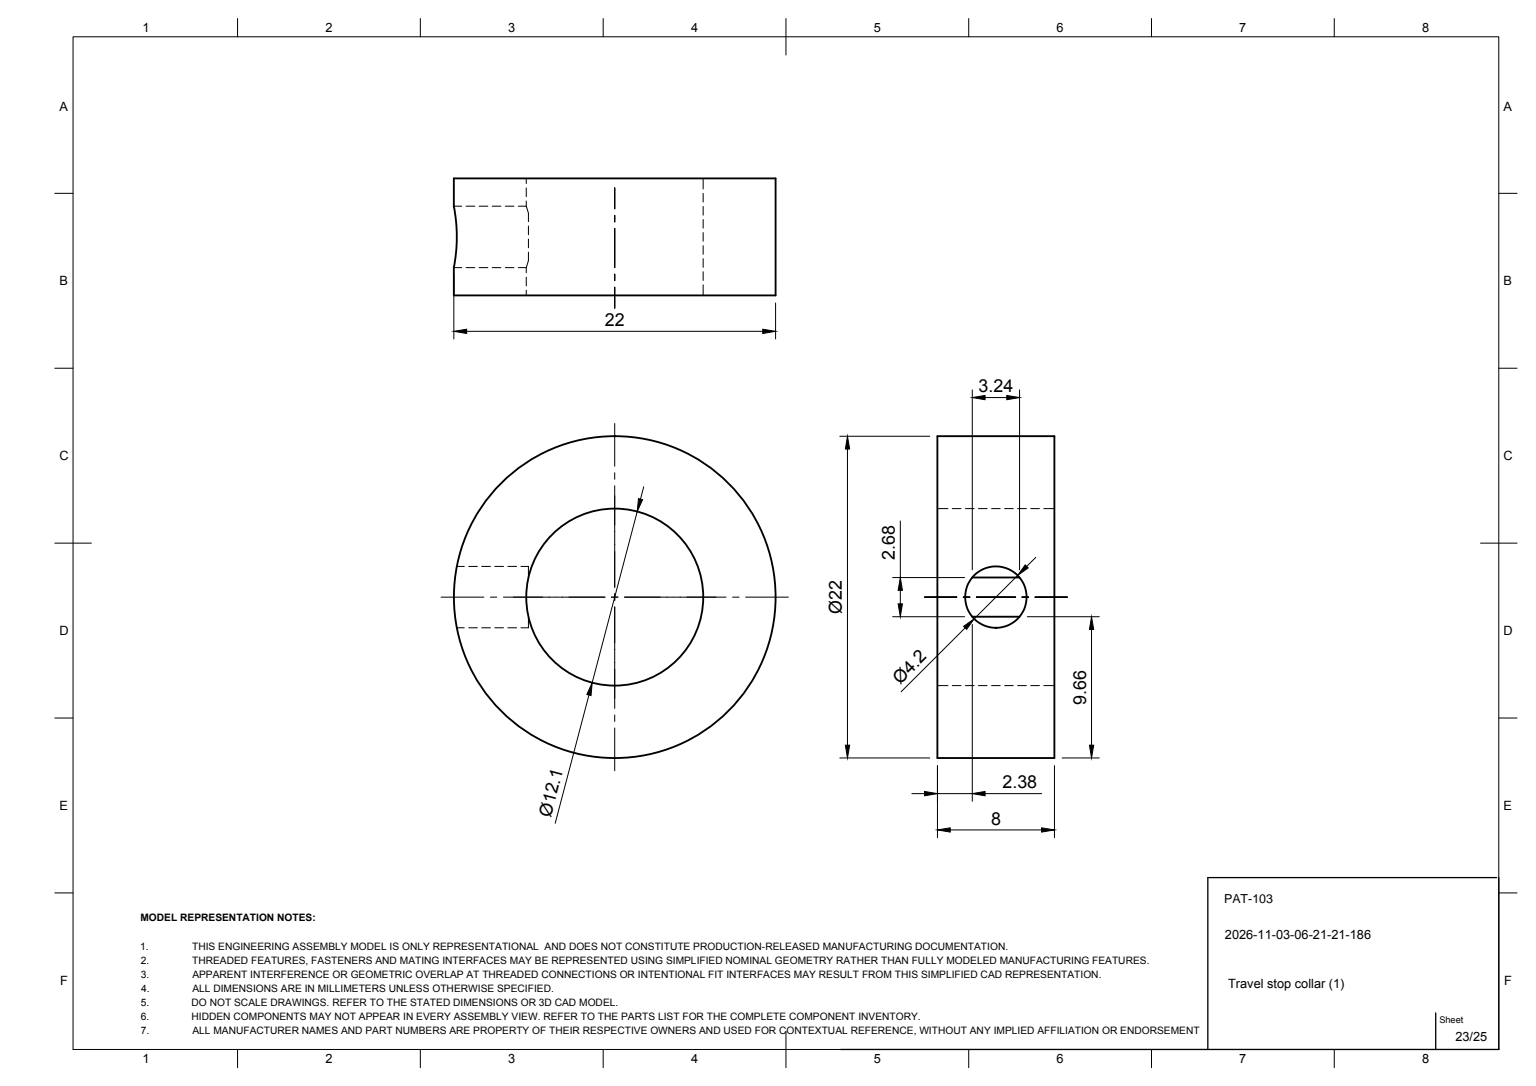
ISO-10303-21;
HEADER;
/* Generated by software containing ST-Developer
 * from STEP Tools, Inc. (www.steptools.com) 
 */

FILE_DESCRIPTION(
/* description */ ('Telescoping shaft support with lock collar'),
/* implementation_level */ '2;1');

FILE_NAME(
/* name */ 'Travel stop collar (1).step',
/* time_stamp */ '2026-10-27T10:48:51-07:00',
/* author */ (''),
/* organization */ (''),
/* preprocessor_version */ 'ST-DEVELOPER v20.2',
/* originating_system */ 'Autodesk Translation Framework v15.17.0.0',
/* authorisation */ '');

FILE_SCHEMA (('AUTOMOTIVE_DESIGN { 1 0 10303 214 3 1 1 }'));
ENDSEC;

DATA;
#10=MECHANICAL_DESIGN_GEOMETRIC_PRESENTATION_REPRESENTATION('',(#256),#7349);
#194=B_SPLINE_CURVE_WITH_KNOTS('',3,(#7006,#7007,#7008,#7009,#7010,#7011),
 .UNSPECIFIED.,.F.,.F.,(4,2,4),(0.81808890434917,0.878131747417167,0.957937926194039),
 .UNSPECIFIED.);
#195=B_SPLINE_CURVE_WITH_KNOTS('',3,(#7015,#7016,#7017,#7018,#7019,#7020),
 .UNSPECIFIED.,.F.,.F.,(4,2,4),(0.31931264206468,0.399118820841551,0.459161663909546),
 .UNSPECIFIED.);
#196=B_SPLINE_CURVE_WITH_KNOTS('',3,(#7021,#7022,#7023,#7024,#7025,#7026),
 .UNSPECIFIED.,.F.,.F.,(4,2,4),(0.179463620219813,0.239506463287808,0.31931264206468),
 .UNSPECIFIED.);
#197=B_SPLINE_CURVE_WITH_KNOTS('',3,(#7027,#7028,#7029,#7030,#7031,#7032),
 .UNSPECIFIED.,.F.,.F.,(4,2,4),(0.957937926194039,1.03774410497091,1.09778694803891),
 .UNSPECIFIED.);
#198=B_SPLINE_CURVE_WITH_KNOTS('',3,(#7036,#7037,#7038,#7039,#7040,#7041,
#7042,#7043,#7044,#7045),.UNSPECIFIED.,.F.,.F.,(4,2,2,2,4),(0.,0.0793157643915219,
0.158631528783044,0.23794361593365,0.317255703084256),.UNSPECIFIED.);
#199=B_SPLINE_CURVE_WITH_KNOTS('',3,(#7047,#7048,#7049,#7050,#7051,#7052,
#7053,#7054,#7055,#7056),.UNSPECIFIED.,.F.,.F.,(4,2,2,2,4),(0.951767109252769,
1.03107919640337,1.11039128355398,1.1897070479455,1.26902281233703),
 .UNSPECIFIED.);
#200=B_SPLINE_CURVE_WITH_KNOTS('',3,(#7057,#7058,#7059,#7060,#7061,#7062,
#7063,#7064,#7065,#7066,#7067,#7068,#7069,#7070,#7071,#7072,#7073,#7074),
 .UNSPECIFIED.,.F.,.F.,(4,2,2,2,2,2,2,2,4),(0.317255703084256,0.396567790234863,
0.475879877385469,0.555195641776991,0.634511406168513,0.713827170560035,
0.793142934951556,0.872455022102163,0.951767109252769),.UNSPECIFIED.);
#216=SHAPE_REPRESENTATION_RELATIONSHIP('SRR','None',#7460,#236);
#236=ADVANCED_BREP_SHAPE_REPRESENTATION('',(#275),#7344);
#256=STYLED_ITEM('',(#7641),#275);
#275=MANIFOLD_SOLID_BREP('Body1',#3980);
#351=FACE_BOUND('',#976,.T.);
#352=FACE_BOUND('',#978,.T.);
#465=PLANE('',#4587);
#466=PLANE('',#4591);
#467=PLANE('',#4598);
#468=PLANE('',#4599);
#672=FACE_OUTER_BOUND('',#970,.T.);
#673=FACE_OUTER_BOUND('',#971,.T.);
#674=FACE_OUTER_BOUND('',#972,.T.);
#675=FACE_OUTER_BOUND('',#973,.T.);
#676=FACE_OUTER_BOUND('',#974,.T.);
#677=FACE_OUTER_BOUND('',#975,.T.);
#678=FACE_OUTER_BOUND('',#977,.T.);
#970=EDGE_LOOP('',(#3468,#3469));
#971=EDGE_LOOP('',(#3470,#3471,#3472,#3473,#3474,#3475,#3476,#3477,#3478,
#3479,#3480));
#972=EDGE_LOOP('',(#3481,#3482));
#973=EDGE_LOOP('',(#3483,#3484,#3485,#3486,#3487,#3488,#3489,#3490,#3491,
#3492,#3493,#3494));
#974=EDGE_LOOP('',(#3495,#3496,#3497,#3498,#3499,#3500,#3501,#3502,#3503));
#975=EDGE_LOOP('',(#3504));
#976=EDGE_LOOP('',(#3505));
#977=EDGE_LOOP('',(#3506));
#978=EDGE_LOOP('',(#3507));
#1248=LINE('',#7001,#1528);
#1249=LINE('',#7034,#1529);
#1250=LINE('',#7076,#1530);
#1251=LINE('',#7080,#1531);
#1252=LINE('',#7082,#1532);
#1253=LINE('',#7087,#1533);
#1254=LINE('',#7089,#1534);
#1528=VECTOR('',#5690,1.);
#1529=VECTOR('',#5697,0.210000000000001);
#1530=VECTOR('',#5700,1.);
#1531=VECTOR('',#5705,0.605);
#1532=VECTOR('',#5706,0.605);
#1533=VECTOR('',#5713,1.1);
#1534=VECTOR('',#5714,1.1);
#1768=CIRCLE('',#4588,0.210000000000001);
#1769=CIRCLE('',#4590,0.210000000000001);
#1770=CIRCLE('',#4593,0.605);
#1771=CIRCLE('',#4594,0.605);
#1772=CIRCLE('',#4596,1.1);
#1773=CIRCLE('',#4597,1.1);
#2072=VERTEX_POINT('',#6999);
#2073=VERTEX_POINT('',#7000);
#2074=VERTEX_POINT('',#7004);
#2075=VERTEX_POINT('',#7005);
#2076=VERTEX_POINT('',#7012);
#2077=VERTEX_POINT('',#7014);
#2078=VERTEX_POINT('',#7033);
#2079=VERTEX_POINT('',#7035);
#2080=VERTEX_POINT('',#7046);
#2081=VERTEX_POINT('',#7078);
#2082=VERTEX_POINT('',#7081);
#2083=VERTEX_POINT('',#7085);
#2084=VERTEX_POINT('',#7088);
#2546=EDGE_CURVE('',#2072,#2073,#1248,.T.);
#2547=EDGE_CURVE('',#2072,#2073,#1768,.T.);
#2548=EDGE_CURVE('',#2074,#2075,#194,.T.);
#2549=EDGE_CURVE('',#2076,#2074,#1769,.T.);
#2550=EDGE_CURVE('',#2077,#2076,#195,.T.);
#2551=EDGE_CURVE('',#2073,#2077,#196,.T.);
#2552=EDGE_CURVE('',#2075,#2072,#197,.T.);
#2553=EDGE_CURVE('',#2075,#2078,#1249,.T.);
#2554=EDGE_CURVE('',#2079,#2078,#198,.T.);
#2555=EDGE_CURVE('',#2080,#2079,#199,.T.);
#2556=EDGE_CURVE('',#2078,#2080,#200,.T.);
#2557=EDGE_CURVE('',#2076,#2074,#1250,.T.);
#2558=EDGE_CURVE('',#2081,#2081,#1770,.T.);
#2559=EDGE_CURVE('',#2081,#2077,#1251,.T.);
#2560=EDGE_CURVE('',#2075,#2082,#1252,.T.);
#2561=EDGE_CURVE('',#2082,#2082,#1771,.T.);
#2562=EDGE_CURVE('',#2083,#2083,#1772,.T.);
#2563=EDGE_CURVE('',#2083,#2080,#1253,.T.);
#2564=EDGE_CURVE('',#2078,#2084,#1254,.T.);
#2565=EDGE_CURVE('',#2084,#2084,#1773,.T.);
#3468=ORIENTED_EDGE('',*,*,#2546,.F.);
#3469=ORIENTED_EDGE('',*,*,#2547,.T.);
#3470=ORIENTED_EDGE('',*,*,#2548,.F.);
#3471=ORIENTED_EDGE('',*,*,#2549,.F.);
#3472=ORIENTED_EDGE('',*,*,#2550,.F.);
#3473=ORIENTED_EDGE('',*,*,#2551,.F.);
#3474=ORIENTED_EDGE('',*,*,#2547,.F.);
#3475=ORIENTED_EDGE('',*,*,#2552,.F.);
#3476=ORIENTED_EDGE('',*,*,#2553,.T.);
#3477=ORIENTED_EDGE('',*,*,#2554,.F.);
#3478=ORIENTED_EDGE('',*,*,#2555,.F.);
#3479=ORIENTED_EDGE('',*,*,#2556,.F.);
#3480=ORIENTED_EDGE('',*,*,#2553,.F.);
#3481=ORIENTED_EDGE('',*,*,#2557,.F.);
#3482=ORIENTED_EDGE('',*,*,#2549,.T.);
#3483=ORIENTED_EDGE('',*,*,#2558,.F.);
#3484=ORIENTED_EDGE('',*,*,#2559,.T.);
#3485=ORIENTED_EDGE('',*,*,#2550,.T.);
#3486=ORIENTED_EDGE('',*,*,#2557,.T.);
#3487=ORIENTED_EDGE('',*,*,#2548,.T.);
#3488=ORIENTED_EDGE('',*,*,#2560,.T.);
#3489=ORIENTED_EDGE('',*,*,#2561,.T.);
#3490=ORIENTED_EDGE('',*,*,#2560,.F.);
#3491=ORIENTED_EDGE('',*,*,#2552,.T.);
#3492=ORIENTED_EDGE('',*,*,#2546,.T.);
#3493=ORIENTED_EDGE('',*,*,#2551,.T.);
#3494=ORIENTED_EDGE('',*,*,#2559,.F.);
#3495=ORIENTED_EDGE('',*,*,#2562,.F.);
#3496=ORIENTED_EDGE('',*,*,#2563,.T.);
#3497=ORIENTED_EDGE('',*,*,#2555,.T.);
#3498=ORIENTED_EDGE('',*,*,#2554,.T.);
#3499=ORIENTED_EDGE('',*,*,#2564,.T.);
#3500=ORIENTED_EDGE('',*,*,#2565,.T.);
#3501=ORIENTED_EDGE('',*,*,#2564,.F.);
#3502=ORIENTED_EDGE('',*,*,#2556,.T.);
#3503=ORIENTED_EDGE('',*,*,#2563,.F.);
#3504=ORIENTED_EDGE('',*,*,#2562,.T.);
#3505=ORIENTED_EDGE('',*,*,#2558,.T.);
#3506=ORIENTED_EDGE('',*,*,#2565,.F.);
#3507=ORIENTED_EDGE('',*,*,#2561,.F.);
#3727=CYLINDRICAL_SURFACE('',#4589,0.210000000000001);
#3728=CYLINDRICAL_SURFACE('',#4592,0.605);
#3729=CYLINDRICAL_SURFACE('',#4595,1.1);
#3915=ADVANCED_FACE('',(#672),#465,.T.);
#3916=ADVANCED_FACE('',(#673),#3727,.F.);
#3917=ADVANCED_FACE('',(#674),#466,.T.);
#3918=ADVANCED_FACE('',(#675),#3728,.F.);
#3919=ADVANCED_FACE('',(#676),#3729,.T.);
#3920=ADVANCED_FACE('',(#677,#351),#467,.T.);
#3921=ADVANCED_FACE('',(#678,#352),#468,.F.);
#3980=CLOSED_SHELL('',(#3915,#3916,#3917,#3918,#3919,#3920,#3921));
#4586=AXIS2_PLACEMENT_3D('',#6997,#5686,#5687);
#4587=AXIS2_PLACEMENT_3D('',#6998,#5688,#5689);
#4588=AXIS2_PLACEMENT_3D('',#7002,#5691,#5692);
#4589=AXIS2_PLACEMENT_3D('',#7003,#5693,#5694);
#4590=AXIS2_PLACEMENT_3D('',#7013,#5695,#5696);
#4591=AXIS2_PLACEMENT_3D('',#7075,#5698,#5699);
#4592=AXIS2_PLACEMENT_3D('',#7077,#5701,#5702);
#4593=AXIS2_PLACEMENT_3D('',#7079,#5703,#5704);
#4594=AXIS2_PLACEMENT_3D('',#7083,#5707,#5708);
#4595=AXIS2_PLACEMENT_3D('',#7084,#5709,#5710);
#4596=AXIS2_PLACEMENT_3D('',#7086,#5711,#5712);
#4597=AXIS2_PLACEMENT_3D('',#7090,#5715,#5716);
#4598=AXIS2_PLACEMENT_3D('',#7091,#5717,#5718);
#4599=AXIS2_PLACEMENT_3D('',#7092,#5719,#5720);
#5686=DIRECTION('axis',(0.,0.,1.));
#5687=DIRECTION('refdir',(1.,0.,0.));
#5688=DIRECTION('center_axis',(0.,0.,1.));
#5689=DIRECTION('ref_axis',(1.,0.,0.));
#5690=DIRECTION('',(1.,0.,0.));
#5691=DIRECTION('center_axis',(0.,0.,1.));
#5692=DIRECTION('ref_axis',(1.,0.,0.));
#5693=DIRECTION('center_axis',(0.,0.,1.));
#5694=DIRECTION('ref_axis',(1.,0.,0.));
#5695=DIRECTION('center_axis',(0.,0.,1.));
#5696=DIRECTION('ref_axis',(1.,0.,0.));
#5697=DIRECTION('',(0.,0.,1.));
#5698=DIRECTION('center_axis',(0.,0.,1.));
#5699=DIRECTION('ref_axis',(1.,0.,0.));
#5700=DIRECTION('',(-1.,0.,0.));
#5701=DIRECTION('center_axis',(1.,0.,0.));
#5702=DIRECTION('ref_axis',(0.,0.,-1.));
#5703=DIRECTION('center_axis',(-1.,0.,0.));
#5704=DIRECTION('ref_axis',(0.,0.,-1.));
#5705=DIRECTION('',(-1.,0.,0.));
#5706=DIRECTION('',(-1.,0.,0.));
#5707=DIRECTION('center_axis',(-1.,0.,0.));
#5708=DIRECTION('ref_axis',(0.,0.,-1.));
#5709=DIRECTION('center_axis',(1.,0.,0.));
#5710=DIRECTION('ref_axis',(0.,0.,-1.));
#5711=DIRECTION('center_axis',(1.,0.,0.));
#5712=DIRECTION('ref_axis',(0.,0.,-1.));
#5713=DIRECTION('',(-1.,0.,0.));
#5714=DIRECTION('',(-1.,0.,0.));
#5715=DIRECTION('center_axis',(1.,0.,0.));
#5716=DIRECTION('ref_axis',(0.,0.,-1.));
#5717=DIRECTION('center_axis',(1.,0.,0.));
#5718=DIRECTION('ref_axis',(0.,0.,-1.));
#5719=DIRECTION('center_axis',(1.,0.,0.));
#5720=DIRECTION('ref_axis',(0.,0.,-1.));
#6997=CARTESIAN_POINT('',(0.,0.,0.));
#6998=CARTESIAN_POINT('Origin',(11.9,0.,4.09));
#6999=CARTESIAN_POINT('',(11.7382131031264,-0.133884278389959,4.09));
#7000=CARTESIAN_POINT('',(12.0617868968736,-0.133884278389959,4.09));
#7001=CARTESIAN_POINT('',(11.5,-0.133884278389959,4.09));
#7002=CARTESIAN_POINT('Origin',(11.9,0.,4.09));
#7003=CARTESIAN_POINT('Origin',(11.9,0.,4.09));
#7004=CARTESIAN_POINT('',(11.7382131031264,0.133884278389959,4.09));
#7005=CARTESIAN_POINT('',(11.69,-3.02060261508153E-17,4.105));
#7006=CARTESIAN_POINT('Ctrl Pts',(11.7382131031264,0.13388427838996,4.09));
#7007=CARTESIAN_POINT('Ctrl Pts',(11.7252788317824,0.118254395260805,4.09354677224418));
#7008=CARTESIAN_POINT('Ctrl Pts',(11.7142006834126,0.100109787682301,4.09698224789957));
#7009=CARTESIAN_POINT('Ctrl Pts',(11.6953614389456,0.0548298721325195,4.1030741628997));
#7010=CARTESIAN_POINT('Ctrl Pts',(11.69,0.0266020595922904,4.105));
#7011=CARTESIAN_POINT('Ctrl Pts',(11.69,0.,4.105));
#7012=CARTESIAN_POINT('',(12.0617868968736,0.133884278389959,4.09));
#7013=CARTESIAN_POINT('Origin',(11.9,0.,4.09));
#7014=CARTESIAN_POINT('',(12.11,-8.21483760496044E-17,4.105));
#7015=CARTESIAN_POINT('Ctrl Pts',(12.11,-1.45716771982052E-16,4.105));
#7016=CARTESIAN_POINT('Ctrl Pts',(12.11,0.0266020595922903,4.105));
#7017=CARTESIAN_POINT('Ctrl Pts',(12.1046385610544,0.0548298721325195,4.1030741628997));
#7018=CARTESIAN_POINT('Ctrl Pts',(12.0857993165874,0.1001097876823,4.09698224789957));
#7019=CARTESIAN_POINT('Ctrl Pts',(12.0747211682176,0.118254395260803,4.09354677224418));
#7020=CARTESIAN_POINT('Ctrl Pts',(12.0617868968736,0.133884278389959,4.09));
#7021=CARTESIAN_POINT('Ctrl Pts',(12.0617868968736,-0.133884278389959,4.09));
#7022=CARTESIAN_POINT('Ctrl Pts',(12.0747211682176,-0.118254395260804,4.09354677224418));
#7023=CARTESIAN_POINT('Ctrl Pts',(12.0857993165874,-0.1001097876823,4.09698224789957));
#7024=CARTESIAN_POINT('Ctrl Pts',(12.1046385610544,-0.0548298721325195,
4.1030741628997));
#7025=CARTESIAN_POINT('Ctrl Pts',(12.11,-0.0266020595922902,4.105));
#7026=CARTESIAN_POINT('Ctrl Pts',(12.11,2.56739074444567E-16,4.105));
#7027=CARTESIAN_POINT('Ctrl Pts',(11.69,7.63278329429795E-17,4.105));
#7028=CARTESIAN_POINT('Ctrl Pts',(11.69,-0.0266020595922903,4.105));
#7029=CARTESIAN_POINT('Ctrl Pts',(11.6953614389456,-0.0548298721325195,
4.1030741628997));
#7030=CARTESIAN_POINT('Ctrl Pts',(11.7142006834126,-0.1001097876823,4.09698224789957));
#7031=CARTESIAN_POINT('Ctrl Pts',(11.7252788317824,-0.118254395260804,4.09354677224418));
#7032=CARTESIAN_POINT('Ctrl Pts',(11.7382131031264,-0.133884278389959,4.09));
#7033=CARTESIAN_POINT('',(11.69,-2.57175827820945E-17,4.6));
#7034=CARTESIAN_POINT('',(11.69,-2.57175827820945E-17,4.09));
#7035=CARTESIAN_POINT('',(11.9,-0.210000000000001,4.57976849370594));
#7036=CARTESIAN_POINT('Ctrl Pts',(11.9,-0.210000000000001,4.57976849370594));
#7037=CARTESIAN_POINT('Ctrl Pts',(11.8735614118695,-0.210000000000001,4.57976849370594));
#7038=CARTESIAN_POINT('Ctrl Pts',(11.8454062187451,-0.204702922670977,4.58084015664674));
#7039=CARTESIAN_POINT('Ctrl Pts',(11.7936865544587,-0.183251796806355,4.58468313707126));
#7040=CARTESIAN_POINT('Ctrl Pts',(11.7701163292589,-0.167101177357215,4.58739593054622));
#7041=CARTESIAN_POINT('Ctrl Pts',(11.7328996853826,-0.129884533480966,4.59246633289124));
#7042=CARTESIAN_POINT('Ctrl Pts',(11.7167483898366,-0.10631394075729,4.59515738895358));
#7043=CARTESIAN_POINT('Ctrl Pts',(11.6952967734303,-0.0545930033295214,
4.59895039220591));
#7044=CARTESIAN_POINT('Ctrl Pts',(11.69,-0.0264373623835355,4.6));
#7045=CARTESIAN_POINT('Ctrl Pts',(11.69,-3.12250225675825E-17,4.6));
#7046=CARTESIAN_POINT('',(12.11,2.28500467976895E-17,4.6));
#7047=CARTESIAN_POINT('Ctrl Pts',(12.11,1.52655665885959E-16,4.6));
#7048=CARTESIAN_POINT('Ctrl Pts',(12.11,-0.0264373623835353,4.6));
#7049=CARTESIAN_POINT('Ctrl Pts',(12.1047032265697,-0.0545930033295213,
4.59895039220591));
#7050=CARTESIAN_POINT('Ctrl Pts',(12.0832516101634,-0.106313940757289,4.59515738895358));
#7051=CARTESIAN_POINT('Ctrl Pts',(12.0671003146174,-0.129884533480966,4.59246633289124));
#7052=CARTESIAN_POINT('Ctrl Pts',(12.0298836707411,-0.167101177357215,4.58739593054622));
#7053=CARTESIAN_POINT('Ctrl Pts',(12.0063134455413,-0.183251796806355,4.58468313707126));
#7054=CARTESIAN_POINT('Ctrl Pts',(11.9545937812549,-0.204702922670977,4.58084015664674));
#7055=CARTESIAN_POINT('Ctrl Pts',(11.9264385881305,-0.210000000000001,4.57976849370594));
#7056=CARTESIAN_POINT('Ctrl Pts',(11.9,-0.210000000000001,4.57976849370594));
#7057=CARTESIAN_POINT('Ctrl Pts',(11.69,6.59194920871187E-17,4.6));
#7058=CARTESIAN_POINT('Ctrl Pts',(11.69,0.0264373623835355,4.6));
#7059=CARTESIAN_POINT('Ctrl Pts',(11.6952967734303,0.0545930033295213,4.59895039220591));
#7060=CARTESIAN_POINT('Ctrl Pts',(11.7167483898366,0.106313940757289,4.59515738895358));
#7061=CARTESIAN_POINT('Ctrl Pts',(11.7328996853826,0.129884533480966,4.59246633289124));
#7062=CARTESIAN_POINT('Ctrl Pts',(11.7701163292589,0.167101177357215,4.58739593054622));
#7063=CARTESIAN_POINT('Ctrl Pts',(11.7936865544587,0.183251796806355,4.58468313707126));
#7064=CARTESIAN_POINT('Ctrl Pts',(11.8454062187451,0.204702922670977,4.58084015664674));
#7065=CARTESIAN_POINT('Ctrl Pts',(11.8735614118695,0.210000000000001,4.57976849370594));
#7066=CARTESIAN_POINT('Ctrl Pts',(11.9264385881305,0.210000000000001,4.57976849370594));
#7067=CARTESIAN_POINT('Ctrl Pts',(11.9545937812549,0.204702922670977,4.58084015664674));
#7068=CARTESIAN_POINT('Ctrl Pts',(12.0063134455413,0.183251796806355,4.58468313707126));
#7069=CARTESIAN_POINT('Ctrl Pts',(12.0298836707411,0.167101177357215,4.58739593054622));
#7070=CARTESIAN_POINT('Ctrl Pts',(12.0671003146174,0.129884533480966,4.59246633289124));
#7071=CARTESIAN_POINT('Ctrl Pts',(12.0832516101634,0.106313940757289,4.59515738895358));
#7072=CARTESIAN_POINT('Ctrl Pts',(12.1047032265697,0.0545930033295214,4.59895039220591));
#7073=CARTESIAN_POINT('Ctrl Pts',(12.11,0.0264373623835354,4.6));
#7074=CARTESIAN_POINT('Ctrl Pts',(12.11,-4.16333634234434E-17,4.6));
#7075=CARTESIAN_POINT('Origin',(11.9,0.,4.09));
#7076=CARTESIAN_POINT('',(11.5,0.133884278389959,4.09));
#7077=CARTESIAN_POINT('Origin',(11.5,0.,3.5));
#7078=CARTESIAN_POINT('',(12.3,-7.40911313484149E-17,4.105));
#7079=CARTESIAN_POINT('Origin',(12.3,0.,3.5));
#7080=CARTESIAN_POINT('',(11.5,-7.40911313484149E-17,4.105));
#7081=CARTESIAN_POINT('',(11.5,-7.40911313484149E-17,4.105));
#7082=CARTESIAN_POINT('',(11.5,-7.40911313484149E-17,4.105));
#7083=CARTESIAN_POINT('Origin',(11.5,0.,3.5));
#7084=CARTESIAN_POINT('Origin',(11.5,0.,3.5));
#7085=CARTESIAN_POINT('',(12.3,-1.34711147906209E-16,4.6));
#7086=CARTESIAN_POINT('Origin',(12.3,0.,3.5));
#7087=CARTESIAN_POINT('',(11.5,-1.34711147906209E-16,4.6));
#7088=CARTESIAN_POINT('',(11.5,-1.34711147906209E-16,4.6));
#7089=CARTESIAN_POINT('',(11.5,-1.34711147906209E-16,4.6));
#7090=CARTESIAN_POINT('Origin',(11.5,0.,3.5));
#7091=CARTESIAN_POINT('Origin',(12.3,0.,3.5));
#7092=CARTESIAN_POINT('Origin',(11.5,0.,3.5));
#7319=UNCERTAINTY_MEASURE_WITH_UNIT(LENGTH_MEASURE(0.001),#7350,
'DISTANCE_ACCURACY_VALUE',
'Maximum model space distance between geometric entities at asserted c
onnectivities');
#7324=UNCERTAINTY_MEASURE_WITH_UNIT(LENGTH_MEASURE(0.001),#7350,
'DISTANCE_ACCURACY_VALUE',
'Maximum model space distance between geometric entities at asserted c
onnectivities');
#7344=(
GEOMETRIC_REPRESENTATION_CONTEXT(3)
GLOBAL_UNCERTAINTY_ASSIGNED_CONTEXT((#7319))
GLOBAL_UNIT_ASSIGNED_CONTEXT((#7350,#7352,#7353))
REPRESENTATION_CONTEXT('','3D')
);
#7349=(
GEOMETRIC_REPRESENTATION_CONTEXT(3)
GLOBAL_UNCERTAINTY_ASSIGNED_CONTEXT((#7324))
GLOBAL_UNIT_ASSIGNED_CONTEXT((#7350,#7352,#7353))
REPRESENTATION_CONTEXT('','3D')
);
#7350=(
LENGTH_UNIT()
NAMED_UNIT(*)
SI_UNIT(.CENTI.,.METRE.)
);
#7352=(
NAMED_UNIT(*)
PLANE_ANGLE_UNIT()
SI_UNIT($,.RADIAN.)
);
#7353=(
NAMED_UNIT(*)
SI_UNIT($,.STERADIAN.)
SOLID_ANGLE_UNIT()
);
#7373=SHAPE_DEFINITION_REPRESENTATION(#7399,#7460);
#7399=PRODUCT_DEFINITION_SHAPE('',$,#7485);
#7460=SHAPE_REPRESENTATION('',(#4586),#7344);
#7465=PRODUCT_DEFINITION_CONTEXT('part definition',#7539,'design');
#7485=PRODUCT_DEFINITION('Travel stop collar (1)',
'Travel stop collar (1)',#7509,#7465);
#7509=PRODUCT_DEFINITION_FORMATION('',$,#7560);
#7539=APPLICATION_CONTEXT(
'Core Data for Automotive Mechanical Design Process');
#7540=PRODUCT_CONTEXT('part definition',#7539,'mechanical');
#7560=PRODUCT('Travel stop collar (1)','Travel stop collar (1)',
'Travel stop collar (1)',(#7540));
#7635=COLOUR_RGB('Off White',0.89,0.88,0.83);
#7636=FILL_AREA_STYLE_COLOUR('',#7635);
#7637=FILL_AREA_STYLE('',(#7636));
#7638=SURFACE_STYLE_FILL_AREA(#7637);
#7639=SURFACE_SIDE_STYLE('',(#7638));
#7640=SURFACE_STYLE_USAGE(.BOTH.,#7639);
#7641=PRESENTATION_STYLE_ASSIGNMENT((#7640));
ENDSEC;
END-ISO-10303-21;
